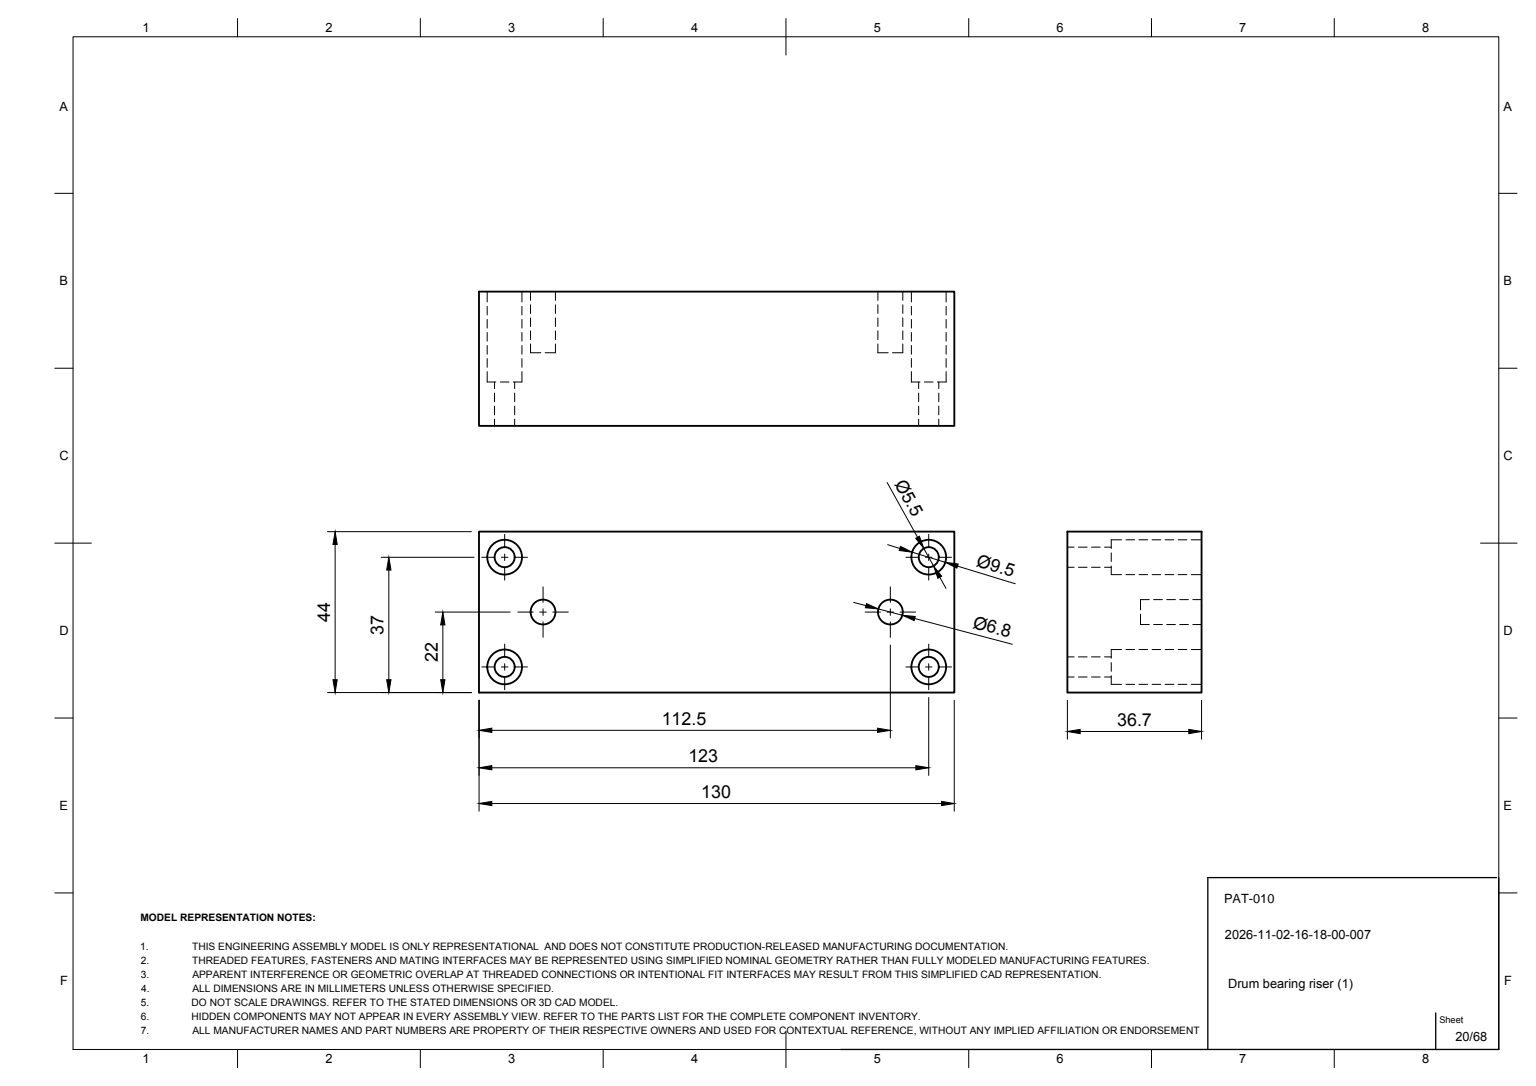
ISO-10303-21;
HEADER;
/* Generated by software containing ST-Developer
 * from STEP Tools, Inc. (www.steptools.com) 
 */

FILE_DESCRIPTION(
/* description */ ('Belt conveyor head drive unit'),
/* implementation_level */ '2;1');

FILE_NAME(
/* name */ 'Drum bearing riser (1).step',
/* time_stamp */ '2026-10-28T03:26:19-07:00',
/* author */ (''),
/* organization */ (''),
/* preprocessor_version */ 'ST-DEVELOPER v20.2',
/* originating_system */ 'Autodesk Translation Framework v15.17.0.0',
/* authorisation */ '');

FILE_SCHEMA (('AUTOMOTIVE_DESIGN { 1 0 10303 214 3 1 1 }'));
ENDSEC;

DATA;
#10=MECHANICAL_DESIGN_GEOMETRIC_PRESENTATION_REPRESENTATION('',(#866),#27069);
#728=SHAPE_REPRESENTATION_RELATIONSHIP('SRR','None',#27372,#797);
#797=ADVANCED_BREP_SHAPE_REPRESENTATION('',(#951),#27014);
#866=STYLED_ITEM('',(#27797),#951);
#951=MANIFOLD_SOLID_BREP('Body1',#13731);
#1111=FACE_BOUND('',#2762,.T.);
#1112=FACE_BOUND('',#2766,.T.);
#1113=FACE_BOUND('',#2770,.T.);
#1114=FACE_BOUND('',#2774,.T.);
#1115=FACE_BOUND('',#2785,.T.);
#1116=FACE_BOUND('',#2786,.T.);
#1117=FACE_BOUND('',#2787,.T.);
#1118=FACE_BOUND('',#2788,.T.);
#1119=FACE_BOUND('',#2789,.T.);
#1120=FACE_BOUND('',#2790,.T.);
#1121=FACE_BOUND('',#2792,.T.);
#1122=FACE_BOUND('',#2793,.T.);
#1123=FACE_BOUND('',#2794,.T.);
#1124=FACE_BOUND('',#2795,.T.);
#1389=PLANE('',#15059);
#1390=PLANE('',#15066);
#1391=PLANE('',#15073);
#1392=PLANE('',#15080);
#1393=PLANE('',#15087);
#1394=PLANE('',#15091);
#1395=PLANE('',#15092);
#1396=PLANE('',#15093);
#1397=PLANE('',#15094);
#1398=PLANE('',#15095);
#1399=PLANE('',#15096);
#1400=PLANE('',#15097);
#1861=FACE_OUTER_BOUND('',#2760,.T.);
#1862=FACE_OUTER_BOUND('',#2761,.T.);
#1863=FACE_OUTER_BOUND('',#2763,.T.);
#1864=FACE_OUTER_BOUND('',#2764,.T.);
#1865=FACE_OUTER_BOUND('',#2765,.T.);
#1866=FACE_OUTER_BOUND('',#2767,.T.);
#1867=FACE_OUTER_BOUND('',#2768,.T.);
#1868=FACE_OUTER_BOUND('',#2769,.T.);
#1869=FACE_OUTER_BOUND('',#2771,.T.);
#1870=FACE_OUTER_BOUND('',#2772,.T.);
#1871=FACE_OUTER_BOUND('',#2773,.T.);
#1872=FACE_OUTER_BOUND('',#2775,.T.);
#1873=FACE_OUTER_BOUND('',#2776,.T.);
#1874=FACE_OUTER_BOUND('',#2777,.T.);
#1875=FACE_OUTER_BOUND('',#2778,.T.);
#1876=FACE_OUTER_BOUND('',#2779,.T.);
#1877=FACE_OUTER_BOUND('',#2780,.T.);
#1878=FACE_OUTER_BOUND('',#2781,.T.);
#1879=FACE_OUTER_BOUND('',#2782,.T.);
#1880=FACE_OUTER_BOUND('',#2783,.T.);
#1881=FACE_OUTER_BOUND('',#2784,.T.);
#1882=FACE_OUTER_BOUND('',#2791,.T.);
#2760=EDGE_LOOP('',(#9972,#9973,#9974,#9975));
#2761=EDGE_LOOP('',(#9976));
#2762=EDGE_LOOP('',(#9977));
#2763=EDGE_LOOP('',(#9978,#9979,#9980,#9981));
#2764=EDGE_LOOP('',(#9982,#9983,#9984,#9985));
#2765=EDGE_LOOP('',(#9986));
#2766=EDGE_LOOP('',(#9987));
#2767=EDGE_LOOP('',(#9988,#9989,#9990,#9991));
#2768=EDGE_LOOP('',(#9992,#9993,#9994,#9995));
#2769=EDGE_LOOP('',(#9996));
#2770=EDGE_LOOP('',(#9997));
#2771=EDGE_LOOP('',(#9998,#9999,#10000,#10001));
#2772=EDGE_LOOP('',(#10002,#10003,#10004,#10005));
#2773=EDGE_LOOP('',(#10006));
#2774=EDGE_LOOP('',(#10007));
#2775=EDGE_LOOP('',(#10008,#10009,#10010,#10011));
#2776=EDGE_LOOP('',(#10012,#10013,#10014,#10015));
#2777=EDGE_LOOP('',(#10016));
#2778=EDGE_LOOP('',(#10017,#10018,#10019,#10020));
#2779=EDGE_LOOP('',(#10021));
#2780=EDGE_LOOP('',(#10022,#10023,#10024,#10025));
#2781=EDGE_LOOP('',(#10026,#10027,#10028,#10029));
#2782=EDGE_LOOP('',(#10030,#10031,#10032,#10033));
#2783=EDGE_LOOP('',(#10034,#10035,#10036,#10037));
#2784=EDGE_LOOP('',(#10038,#10039,#10040,#10041));
#2785=EDGE_LOOP('',(#10042));
#2786=EDGE_LOOP('',(#10043));
#2787=EDGE_LOOP('',(#10044));
#2788=EDGE_LOOP('',(#10045));
#2789=EDGE_LOOP('',(#10046));
#2790=EDGE_LOOP('',(#10047));
#2791=EDGE_LOOP('',(#10048,#10049,#10050,#10051));
#2792=EDGE_LOOP('',(#10052));
#2793=EDGE_LOOP('',(#10053));
#2794=EDGE_LOOP('',(#10054));
#2795=EDGE_LOOP('',(#10055));
#3761=LINE('',#22069,#4553);
#3762=LINE('',#22077,#4554);
#3763=LINE('',#22082,#4555);
#3764=LINE('',#22090,#4556);
#3765=LINE('',#22095,#4557);
#3766=LINE('',#22103,#4558);
#3767=LINE('',#22108,#4559);
#3768=LINE('',#22116,#4560);
#3769=LINE('',#22121,#4561);
#3770=LINE('',#22128,#4562);
#3771=LINE('',#22134,#4563);
#3772=LINE('',#22136,#4564);
#3773=LINE('',#22138,#4565);
#3774=LINE('',#22139,#4566);
#3775=LINE('',#22142,#4567);
#3776=LINE('',#22144,#4568);
#3777=LINE('',#22145,#4569);
#3778=LINE('',#22148,#4570);
#3779=LINE('',#22150,#4571);
#3780=LINE('',#22151,#4572);
#3781=LINE('',#22153,#4573);
#3782=LINE('',#22154,#4574);
#4553=VECTOR('',#17689,0.475);
#4554=VECTOR('',#17700,0.275);
#4555=VECTOR('',#17705,0.475);
#4556=VECTOR('',#17716,0.275);
#4557=VECTOR('',#17721,0.475);
#4558=VECTOR('',#17732,0.275);
#4559=VECTOR('',#17737,0.475);
#4560=VECTOR('',#17748,0.275);
#4561=VECTOR('',#17753,0.34);
#4562=VECTOR('',#17762,0.34);
#4563=VECTOR('',#17769,1.);
#4564=VECTOR('',#17770,1.);
#4565=VECTOR('',#17771,1.);
#4566=VECTOR('',#17772,1.);
#4567=VECTOR('',#17775,1.);
#4568=VECTOR('',#17776,1.);
#4569=VECTOR('',#17777,1.);
#4570=VECTOR('',#17780,1.);
#4571=VECTOR('',#17781,1.);
#4572=VECTOR('',#17782,1.);
#4573=VECTOR('',#17785,1.);
#4574=VECTOR('',#17786,1.);
#5326=CIRCLE('',#15057,0.475);
#5327=CIRCLE('',#15058,0.475);
#5328=CIRCLE('',#15060,0.275);
#5329=CIRCLE('',#15062,0.275);
#5330=CIRCLE('',#15064,0.475);
#5331=CIRCLE('',#15065,0.475);
#5332=CIRCLE('',#15067,0.275);
#5333=CIRCLE('',#15069,0.275);
#5334=CIRCLE('',#15071,0.475);
#5335=CIRCLE('',#15072,0.475);
#5336=CIRCLE('',#15074,0.275);
#5337=CIRCLE('',#15076,0.275);
#5338=CIRCLE('',#15078,0.475);
#5339=CIRCLE('',#15079,0.475);
#5340=CIRCLE('',#15081,0.275);
#5341=CIRCLE('',#15083,0.275);
#5342=CIRCLE('',#15085,0.34);
#5343=CIRCLE('',#15086,0.34);
#5344=CIRCLE('',#15089,0.34);
#5345=CIRCLE('',#15090,0.34);
#6291=VERTEX_POINT('',#22066);
#6292=VERTEX_POINT('',#22068);
#6293=VERTEX_POINT('',#22072);
#6294=VERTEX_POINT('',#22075);
#6295=VERTEX_POINT('',#22079);
#6296=VERTEX_POINT('',#22081);
#6297=VERTEX_POINT('',#22085);
#6298=VERTEX_POINT('',#22088);
#6299=VERTEX_POINT('',#22092);
#6300=VERTEX_POINT('',#22094);
#6301=VERTEX_POINT('',#22098);
#6302=VERTEX_POINT('',#22101);
#6303=VERTEX_POINT('',#22105);
#6304=VERTEX_POINT('',#22107);
#6305=VERTEX_POINT('',#22111);
#6306=VERTEX_POINT('',#22114);
#6307=VERTEX_POINT('',#22118);
#6308=VERTEX_POINT('',#22120);
#6309=VERTEX_POINT('',#22125);
#6310=VERTEX_POINT('',#22127);
#6311=VERTEX_POINT('',#22132);
#6312=VERTEX_POINT('',#22133);
#6313=VERTEX_POINT('',#22135);
#6314=VERTEX_POINT('',#22137);
#6315=VERTEX_POINT('',#22141);
#6316=VERTEX_POINT('',#22143);
#6317=VERTEX_POINT('',#22147);
#6318=VERTEX_POINT('',#22149);
#7678=EDGE_CURVE('',#6291,#6291,#5326,.T.);
#7679=EDGE_CURVE('',#6291,#6292,#3761,.T.);
#7680=EDGE_CURVE('',#6292,#6292,#5327,.T.);
#7681=EDGE_CURVE('',#6293,#6293,#5328,.T.);
#7682=EDGE_CURVE('',#6294,#6294,#5329,.T.);
#7683=EDGE_CURVE('',#6294,#6293,#3762,.T.);
#7684=EDGE_CURVE('',#6295,#6295,#5330,.T.);
#7685=EDGE_CURVE('',#6295,#6296,#3763,.T.);
#7686=EDGE_CURVE('',#6296,#6296,#5331,.T.);
#7687=EDGE_CURVE('',#6297,#6297,#5332,.T.);
#7688=EDGE_CURVE('',#6298,#6298,#5333,.T.);
#7689=EDGE_CURVE('',#6298,#6297,#3764,.T.);
#7690=EDGE_CURVE('',#6299,#6299,#5334,.T.);
#7691=EDGE_CURVE('',#6299,#6300,#3765,.T.);
#7692=EDGE_CURVE('',#6300,#6300,#5335,.T.);
#7693=EDGE_CURVE('',#6301,#6301,#5336,.T.);
#7694=EDGE_CURVE('',#6302,#6302,#5337,.T.);
#7695=EDGE_CURVE('',#6302,#6301,#3766,.T.);
#7696=EDGE_CURVE('',#6303,#6303,#5338,.T.);
#7697=EDGE_CURVE('',#6303,#6304,#3767,.T.);
#7698=EDGE_CURVE('',#6304,#6304,#5339,.T.);
#7699=EDGE_CURVE('',#6305,#6305,#5340,.T.);
#7700=EDGE_CURVE('',#6306,#6306,#5341,.T.);
#7701=EDGE_CURVE('',#6306,#6305,#3768,.T.);
#7702=EDGE_CURVE('',#6307,#6307,#5342,.T.);
#7703=EDGE_CURVE('',#6307,#6308,#3769,.T.);
#7704=EDGE_CURVE('',#6308,#6308,#5343,.T.);
#7705=EDGE_CURVE('',#6309,#6309,#5344,.T.);
#7706=EDGE_CURVE('',#6309,#6310,#3770,.T.);
#7707=EDGE_CURVE('',#6310,#6310,#5345,.T.);
#7708=EDGE_CURVE('',#6311,#6312,#3771,.T.);
#7709=EDGE_CURVE('',#6312,#6313,#3772,.T.);
#7710=EDGE_CURVE('',#6314,#6313,#3773,.T.);
#7711=EDGE_CURVE('',#6311,#6314,#3774,.T.);
#7712=EDGE_CURVE('',#6315,#6311,#3775,.T.);
#7713=EDGE_CURVE('',#6316,#6314,#3776,.T.);
#7714=EDGE_CURVE('',#6315,#6316,#3777,.T.);
#7715=EDGE_CURVE('',#6317,#6315,#3778,.T.);
#7716=EDGE_CURVE('',#6318,#6316,#3779,.T.);
#7717=EDGE_CURVE('',#6317,#6318,#3780,.T.);
#7718=EDGE_CURVE('',#6312,#6317,#3781,.T.);
#7719=EDGE_CURVE('',#6313,#6318,#3782,.T.);
#9972=ORIENTED_EDGE('',*,*,#7678,.F.);
#9973=ORIENTED_EDGE('',*,*,#7679,.T.);
#9974=ORIENTED_EDGE('',*,*,#7680,.F.);
#9975=ORIENTED_EDGE('',*,*,#7679,.F.);
#9976=ORIENTED_EDGE('',*,*,#7678,.T.);
#9977=ORIENTED_EDGE('',*,*,#7681,.F.);
#9978=ORIENTED_EDGE('',*,*,#7682,.F.);
#9979=ORIENTED_EDGE('',*,*,#7683,.T.);
#9980=ORIENTED_EDGE('',*,*,#7681,.T.);
#9981=ORIENTED_EDGE('',*,*,#7683,.F.);
#9982=ORIENTED_EDGE('',*,*,#7684,.F.);
#9983=ORIENTED_EDGE('',*,*,#7685,.T.);
#9984=ORIENTED_EDGE('',*,*,#7686,.F.);
#9985=ORIENTED_EDGE('',*,*,#7685,.F.);
#9986=ORIENTED_EDGE('',*,*,#7684,.T.);
#9987=ORIENTED_EDGE('',*,*,#7687,.F.);
#9988=ORIENTED_EDGE('',*,*,#7688,.F.);
#9989=ORIENTED_EDGE('',*,*,#7689,.T.);
#9990=ORIENTED_EDGE('',*,*,#7687,.T.);
#9991=ORIENTED_EDGE('',*,*,#7689,.F.);
#9992=ORIENTED_EDGE('',*,*,#7690,.F.);
#9993=ORIENTED_EDGE('',*,*,#7691,.T.);
#9994=ORIENTED_EDGE('',*,*,#7692,.F.);
#9995=ORIENTED_EDGE('',*,*,#7691,.F.);
#9996=ORIENTED_EDGE('',*,*,#7690,.T.);
#9997=ORIENTED_EDGE('',*,*,#7693,.F.);
#9998=ORIENTED_EDGE('',*,*,#7694,.F.);
#9999=ORIENTED_EDGE('',*,*,#7695,.T.);
#10000=ORIENTED_EDGE('',*,*,#7693,.T.);
#10001=ORIENTED_EDGE('',*,*,#7695,.F.);
#10002=ORIENTED_EDGE('',*,*,#7696,.F.);
#10003=ORIENTED_EDGE('',*,*,#7697,.T.);
#10004=ORIENTED_EDGE('',*,*,#7698,.F.);
#10005=ORIENTED_EDGE('',*,*,#7697,.F.);
#10006=ORIENTED_EDGE('',*,*,#7696,.T.);
#10007=ORIENTED_EDGE('',*,*,#7699,.F.);
#10008=ORIENTED_EDGE('',*,*,#7700,.F.);
#10009=ORIENTED_EDGE('',*,*,#7701,.T.);
#10010=ORIENTED_EDGE('',*,*,#7699,.T.);
#10011=ORIENTED_EDGE('',*,*,#7701,.F.);
#10012=ORIENTED_EDGE('',*,*,#7702,.F.);
#10013=ORIENTED_EDGE('',*,*,#7703,.T.);
#10014=ORIENTED_EDGE('',*,*,#7704,.F.);
#10015=ORIENTED_EDGE('',*,*,#7703,.F.);
#10016=ORIENTED_EDGE('',*,*,#7702,.T.);
#10017=ORIENTED_EDGE('',*,*,#7705,.F.);
#10018=ORIENTED_EDGE('',*,*,#7706,.T.);
#10019=ORIENTED_EDGE('',*,*,#7707,.F.);
#10020=ORIENTED_EDGE('',*,*,#7706,.F.);
#10021=ORIENTED_EDGE('',*,*,#7705,.T.);
#10022=ORIENTED_EDGE('',*,*,#7708,.T.);
#10023=ORIENTED_EDGE('',*,*,#7709,.T.);
#10024=ORIENTED_EDGE('',*,*,#7710,.F.);
#10025=ORIENTED_EDGE('',*,*,#7711,.F.);
#10026=ORIENTED_EDGE('',*,*,#7712,.T.);
#10027=ORIENTED_EDGE('',*,*,#7711,.T.);
#10028=ORIENTED_EDGE('',*,*,#7713,.F.);
#10029=ORIENTED_EDGE('',*,*,#7714,.F.);
#10030=ORIENTED_EDGE('',*,*,#7715,.T.);
#10031=ORIENTED_EDGE('',*,*,#7714,.T.);
#10032=ORIENTED_EDGE('',*,*,#7716,.F.);
#10033=ORIENTED_EDGE('',*,*,#7717,.F.);
#10034=ORIENTED_EDGE('',*,*,#7718,.T.);
#10035=ORIENTED_EDGE('',*,*,#7717,.T.);
#10036=ORIENTED_EDGE('',*,*,#7719,.F.);
#10037=ORIENTED_EDGE('',*,*,#7709,.F.);
#10038=ORIENTED_EDGE('',*,*,#7719,.T.);
#10039=ORIENTED_EDGE('',*,*,#7716,.T.);
#10040=ORIENTED_EDGE('',*,*,#7713,.T.);
#10041=ORIENTED_EDGE('',*,*,#7710,.T.);
#10042=ORIENTED_EDGE('',*,*,#7680,.T.);
#10043=ORIENTED_EDGE('',*,*,#7686,.T.);
#10044=ORIENTED_EDGE('',*,*,#7692,.T.);
#10045=ORIENTED_EDGE('',*,*,#7698,.T.);
#10046=ORIENTED_EDGE('',*,*,#7704,.T.);
#10047=ORIENTED_EDGE('',*,*,#7707,.T.);
#10048=ORIENTED_EDGE('',*,*,#7718,.F.);
#10049=ORIENTED_EDGE('',*,*,#7708,.F.);
#10050=ORIENTED_EDGE('',*,*,#7712,.F.);
#10051=ORIENTED_EDGE('',*,*,#7715,.F.);
#10052=ORIENTED_EDGE('',*,*,#7682,.T.);
#10053=ORIENTED_EDGE('',*,*,#7688,.T.);
#10054=ORIENTED_EDGE('',*,*,#7694,.T.);
#10055=ORIENTED_EDGE('',*,*,#7700,.T.);
#12648=CYLINDRICAL_SURFACE('',#15056,0.475);
#12649=CYLINDRICAL_SURFACE('',#15061,0.275);
#12650=CYLINDRICAL_SURFACE('',#15063,0.475);
#12651=CYLINDRICAL_SURFACE('',#15068,0.275);
#12652=CYLINDRICAL_SURFACE('',#15070,0.475);
#12653=CYLINDRICAL_SURFACE('',#15075,0.275);
#12654=CYLINDRICAL_SURFACE('',#15077,0.475);
#12655=CYLINDRICAL_SURFACE('',#15082,0.275);
#12656=CYLINDRICAL_SURFACE('',#15084,0.34);
#12657=CYLINDRICAL_SURFACE('',#15088,0.34);
#13140=ADVANCED_FACE('',(#1861),#12648,.F.);
#13141=ADVANCED_FACE('',(#1862,#1111),#1389,.T.);
#13142=ADVANCED_FACE('',(#1863),#12649,.F.);
#13143=ADVANCED_FACE('',(#1864),#12650,.F.);
#13144=ADVANCED_FACE('',(#1865,#1112),#1390,.T.);
#13145=ADVANCED_FACE('',(#1866),#12651,.F.);
#13146=ADVANCED_FACE('',(#1867),#12652,.F.);
#13147=ADVANCED_FACE('',(#1868,#1113),#1391,.T.);
#13148=ADVANCED_FACE('',(#1869),#12653,.F.);
#13149=ADVANCED_FACE('',(#1870),#12654,.F.);
#13150=ADVANCED_FACE('',(#1871,#1114),#1392,.T.);
#13151=ADVANCED_FACE('',(#1872),#12655,.F.);
#13152=ADVANCED_FACE('',(#1873),#12656,.F.);
#13153=ADVANCED_FACE('',(#1874),#1393,.T.);
#13154=ADVANCED_FACE('',(#1875),#12657,.F.);
#13155=ADVANCED_FACE('',(#1876),#1394,.T.);
#13156=ADVANCED_FACE('',(#1877),#1395,.T.);
#13157=ADVANCED_FACE('',(#1878),#1396,.T.);
#13158=ADVANCED_FACE('',(#1879),#1397,.T.);
#13159=ADVANCED_FACE('',(#1880),#1398,.T.);
#13160=ADVANCED_FACE('',(#1881,#1115,#1116,#1117,#1118,#1119,#1120),#1399,
 .T.);
#13161=ADVANCED_FACE('',(#1882,#1121,#1122,#1123,#1124),#1400,.F.);
#13731=CLOSED_SHELL('',(#13140,#13141,#13142,#13143,#13144,#13145,#13146,
#13147,#13148,#13149,#13150,#13151,#13152,#13153,#13154,#13155,#13156,#13157,
#13158,#13159,#13160,#13161));
#15055=AXIS2_PLACEMENT_3D('',#22064,#17683,#17684);
#15056=AXIS2_PLACEMENT_3D('',#22065,#17685,#17686);
#15057=AXIS2_PLACEMENT_3D('',#22067,#17687,#17688);
#15058=AXIS2_PLACEMENT_3D('',#22070,#17690,#17691);
#15059=AXIS2_PLACEMENT_3D('',#22071,#17692,#17693);
#15060=AXIS2_PLACEMENT_3D('',#22073,#17694,#17695);
#15061=AXIS2_PLACEMENT_3D('',#22074,#17696,#17697);
#15062=AXIS2_PLACEMENT_3D('',#22076,#17698,#17699);
#15063=AXIS2_PLACEMENT_3D('',#22078,#17701,#17702);
#15064=AXIS2_PLACEMENT_3D('',#22080,#17703,#17704);
#15065=AXIS2_PLACEMENT_3D('',#22083,#17706,#17707);
#15066=AXIS2_PLACEMENT_3D('',#22084,#17708,#17709);
#15067=AXIS2_PLACEMENT_3D('',#22086,#17710,#17711);
#15068=AXIS2_PLACEMENT_3D('',#22087,#17712,#17713);
#15069=AXIS2_PLACEMENT_3D('',#22089,#17714,#17715);
#15070=AXIS2_PLACEMENT_3D('',#22091,#17717,#17718);
#15071=AXIS2_PLACEMENT_3D('',#22093,#17719,#17720);
#15072=AXIS2_PLACEMENT_3D('',#22096,#17722,#17723);
#15073=AXIS2_PLACEMENT_3D('',#22097,#17724,#17725);
#15074=AXIS2_PLACEMENT_3D('',#22099,#17726,#17727);
#15075=AXIS2_PLACEMENT_3D('',#22100,#17728,#17729);
#15076=AXIS2_PLACEMENT_3D('',#22102,#17730,#17731);
#15077=AXIS2_PLACEMENT_3D('',#22104,#17733,#17734);
#15078=AXIS2_PLACEMENT_3D('',#22106,#17735,#17736);
#15079=AXIS2_PLACEMENT_3D('',#22109,#17738,#17739);
#15080=AXIS2_PLACEMENT_3D('',#22110,#17740,#17741);
#15081=AXIS2_PLACEMENT_3D('',#22112,#17742,#17743);
#15082=AXIS2_PLACEMENT_3D('',#22113,#17744,#17745);
#15083=AXIS2_PLACEMENT_3D('',#22115,#17746,#17747);
#15084=AXIS2_PLACEMENT_3D('',#22117,#17749,#17750);
#15085=AXIS2_PLACEMENT_3D('',#22119,#17751,#17752);
#15086=AXIS2_PLACEMENT_3D('',#22122,#17754,#17755);
#15087=AXIS2_PLACEMENT_3D('',#22123,#17756,#17757);
#15088=AXIS2_PLACEMENT_3D('',#22124,#17758,#17759);
#15089=AXIS2_PLACEMENT_3D('',#22126,#17760,#17761);
#15090=AXIS2_PLACEMENT_3D('',#22129,#17763,#17764);
#15091=AXIS2_PLACEMENT_3D('',#22130,#17765,#17766);
#15092=AXIS2_PLACEMENT_3D('',#22131,#17767,#17768);
#15093=AXIS2_PLACEMENT_3D('',#22140,#17773,#17774);
#15094=AXIS2_PLACEMENT_3D('',#22146,#17778,#17779);
#15095=AXIS2_PLACEMENT_3D('',#22152,#17783,#17784);
#15096=AXIS2_PLACEMENT_3D('',#22155,#17787,#17788);
#15097=AXIS2_PLACEMENT_3D('',#22156,#17789,#17790);
#17683=DIRECTION('axis',(0.,0.,1.));
#17684=DIRECTION('refdir',(1.,0.,0.));
#17685=DIRECTION('center_axis',(0.,0.,1.));
#17686=DIRECTION('ref_axis',(1.,0.,0.));
#17687=DIRECTION('center_axis',(0.,0.,1.));
#17688=DIRECTION('ref_axis',(1.,0.,0.));
#17689=DIRECTION('',(0.,0.,1.));
#17690=DIRECTION('center_axis',(0.,0.,-1.));
#17691=DIRECTION('ref_axis',(1.,0.,0.));
#17692=DIRECTION('center_axis',(0.,0.,1.));
#17693=DIRECTION('ref_axis',(1.,0.,0.));
#17694=DIRECTION('center_axis',(0.,0.,1.));
#17695=DIRECTION('ref_axis',(1.,0.,0.));
#17696=DIRECTION('center_axis',(0.,0.,1.));
#17697=DIRECTION('ref_axis',(1.,0.,0.));
#17698=DIRECTION('center_axis',(0.,0.,1.));
#17699=DIRECTION('ref_axis',(1.,0.,0.));
#17700=DIRECTION('',(0.,0.,1.));
#17701=DIRECTION('center_axis',(0.,0.,1.));
#17702=DIRECTION('ref_axis',(1.,0.,0.));
#17703=DIRECTION('center_axis',(0.,0.,1.));
#17704=DIRECTION('ref_axis',(1.,0.,0.));
#17705=DIRECTION('',(0.,0.,1.));
#17706=DIRECTION('center_axis',(0.,0.,-1.));
#17707=DIRECTION('ref_axis',(1.,0.,0.));
#17708=DIRECTION('center_axis',(0.,0.,1.));
#17709=DIRECTION('ref_axis',(1.,0.,0.));
#17710=DIRECTION('center_axis',(0.,0.,1.));
#17711=DIRECTION('ref_axis',(1.,0.,0.));
#17712=DIRECTION('center_axis',(0.,0.,1.));
#17713=DIRECTION('ref_axis',(1.,0.,0.));
#17714=DIRECTION('center_axis',(0.,0.,1.));
#17715=DIRECTION('ref_axis',(1.,0.,0.));
#17716=DIRECTION('',(0.,0.,1.));
#17717=DIRECTION('center_axis',(0.,0.,1.));
#17718=DIRECTION('ref_axis',(1.,0.,0.));
#17719=DIRECTION('center_axis',(0.,0.,1.));
#17720=DIRECTION('ref_axis',(1.,0.,0.));
#17721=DIRECTION('',(0.,0.,1.));
#17722=DIRECTION('center_axis',(0.,0.,-1.));
#17723=DIRECTION('ref_axis',(1.,0.,0.));
#17724=DIRECTION('center_axis',(0.,0.,1.));
#17725=DIRECTION('ref_axis',(1.,0.,0.));
#17726=DIRECTION('center_axis',(0.,0.,1.));
#17727=DIRECTION('ref_axis',(1.,0.,0.));
#17728=DIRECTION('center_axis',(0.,0.,1.));
#17729=DIRECTION('ref_axis',(1.,0.,0.));
#17730=DIRECTION('center_axis',(0.,0.,1.));
#17731=DIRECTION('ref_axis',(1.,0.,0.));
#17732=DIRECTION('',(0.,0.,1.));
#17733=DIRECTION('center_axis',(0.,0.,1.));
#17734=DIRECTION('ref_axis',(1.,0.,0.));
#17735=DIRECTION('center_axis',(0.,0.,1.));
#17736=DIRECTION('ref_axis',(1.,0.,0.));
#17737=DIRECTION('',(0.,0.,1.));
#17738=DIRECTION('center_axis',(0.,0.,-1.));
#17739=DIRECTION('ref_axis',(1.,0.,0.));
#17740=DIRECTION('center_axis',(0.,0.,1.));
#17741=DIRECTION('ref_axis',(1.,0.,0.));
#17742=DIRECTION('center_axis',(0.,0.,1.));
#17743=DIRECTION('ref_axis',(1.,0.,0.));
#17744=DIRECTION('center_axis',(0.,0.,1.));
#17745=DIRECTION('ref_axis',(1.,0.,0.));
#17746=DIRECTION('center_axis',(0.,0.,1.));
#17747=DIRECTION('ref_axis',(1.,0.,0.));
#17748=DIRECTION('',(0.,0.,1.));
#17749=DIRECTION('center_axis',(0.,0.,1.));
#17750=DIRECTION('ref_axis',(1.,0.,0.));
#17751=DIRECTION('center_axis',(0.,0.,1.));
#17752=DIRECTION('ref_axis',(1.,0.,0.));
#17753=DIRECTION('',(0.,0.,1.));
#17754=DIRECTION('center_axis',(0.,0.,-1.));
#17755=DIRECTION('ref_axis',(1.,0.,0.));
#17756=DIRECTION('center_axis',(0.,0.,1.));
#17757=DIRECTION('ref_axis',(1.,0.,0.));
#17758=DIRECTION('center_axis',(0.,0.,1.));
#17759=DIRECTION('ref_axis',(1.,0.,0.));
#17760=DIRECTION('center_axis',(0.,0.,1.));
#17761=DIRECTION('ref_axis',(1.,0.,0.));
#17762=DIRECTION('',(0.,0.,1.));
#17763=DIRECTION('center_axis',(0.,0.,-1.));
#17764=DIRECTION('ref_axis',(1.,0.,0.));
#17765=DIRECTION('center_axis',(0.,0.,1.));
#17766=DIRECTION('ref_axis',(1.,0.,0.));
#17767=DIRECTION('center_axis',(0.,1.,0.));
#17768=DIRECTION('ref_axis',(-1.,0.,0.));
#17769=DIRECTION('',(-1.,0.,0.));
#17770=DIRECTION('',(0.,0.,1.));
#17771=DIRECTION('',(-1.,0.,0.));
#17772=DIRECTION('',(0.,0.,1.));
#17773=DIRECTION('center_axis',(1.,0.,0.));
#17774=DIRECTION('ref_axis',(0.,1.,0.));
#17775=DIRECTION('',(0.,1.,0.));
#17776=DIRECTION('',(0.,1.,0.));
#17777=DIRECTION('',(0.,0.,1.));
#17778=DIRECTION('center_axis',(0.,-1.,0.));
#17779=DIRECTION('ref_axis',(1.,0.,0.));
#17780=DIRECTION('',(1.,0.,0.));
#17781=DIRECTION('',(1.,0.,0.));
#17782=DIRECTION('',(0.,0.,1.));
#17783=DIRECTION('center_axis',(-1.,0.,0.));
#17784=DIRECTION('ref_axis',(0.,-1.,0.));
#17785=DIRECTION('',(0.,-1.,0.));
#17786=DIRECTION('',(0.,-1.,0.));
#17787=DIRECTION('center_axis',(0.,0.,1.));
#17788=DIRECTION('ref_axis',(1.,0.,0.));
#17789=DIRECTION('center_axis',(0.,0.,1.));
#17790=DIRECTION('ref_axis',(1.,0.,0.));
#22064=CARTESIAN_POINT('',(0.,0.,0.));
#22065=CARTESIAN_POINT('Origin',(12.7709100301812,41.5,1.2));
#22066=CARTESIAN_POINT('',(12.2959100301812,41.5,1.2));
#22067=CARTESIAN_POINT('Origin',(12.7709100301812,41.5,1.2));
#22068=CARTESIAN_POINT('',(12.2959100301812,41.5,3.67));
#22069=CARTESIAN_POINT('',(12.2959100301812,41.5,1.2));
#22070=CARTESIAN_POINT('Origin',(12.7709100301812,41.5,3.67));
#22071=CARTESIAN_POINT('Origin',(12.7709100301812,41.5,1.2));
#22072=CARTESIAN_POINT('',(12.4959100301812,41.5,1.2));
#22073=CARTESIAN_POINT('Origin',(12.7709100301812,41.5,1.2));
#22074=CARTESIAN_POINT('Origin',(12.7709100301812,41.5,-0.1));
#22075=CARTESIAN_POINT('',(12.4959100301812,41.5,0.));
#22076=CARTESIAN_POINT('Origin',(12.7709100301812,41.5,0.));
#22077=CARTESIAN_POINT('',(12.4959100301812,41.5,-0.1));
#22078=CARTESIAN_POINT('Origin',(12.7709100301812,38.5,1.2));
#22079=CARTESIAN_POINT('',(12.2959100301812,38.5,1.2));
#22080=CARTESIAN_POINT('Origin',(12.7709100301812,38.5,1.2));
#22081=CARTESIAN_POINT('',(12.2959100301812,38.5,3.67));
#22082=CARTESIAN_POINT('',(12.2959100301812,38.5,1.2));
#22083=CARTESIAN_POINT('Origin',(12.7709100301812,38.5,3.67));
#22084=CARTESIAN_POINT('Origin',(12.7709100301812,38.5,1.2));
#22085=CARTESIAN_POINT('',(12.4959100301812,38.5,1.2));
#22086=CARTESIAN_POINT('Origin',(12.7709100301812,38.5,1.2));
#22087=CARTESIAN_POINT('Origin',(12.7709100301812,38.5,-0.1));
#22088=CARTESIAN_POINT('',(12.4959100301812,38.5,0.));
#22089=CARTESIAN_POINT('Origin',(12.7709100301812,38.5,0.));
#22090=CARTESIAN_POINT('',(12.4959100301812,38.5,-0.1));
#22091=CARTESIAN_POINT('Origin',(1.17091003018116,41.5,1.2));
#22092=CARTESIAN_POINT('',(0.695910030181156,41.5,1.2));
#22093=CARTESIAN_POINT('Origin',(1.17091003018116,41.5,1.2));
#22094=CARTESIAN_POINT('',(0.695910030181156,41.5,3.67));
#22095=CARTESIAN_POINT('',(0.695910030181156,41.5,1.2));
#22096=CARTESIAN_POINT('Origin',(1.17091003018116,41.5,3.67));
#22097=CARTESIAN_POINT('Origin',(1.17091003018116,41.5,1.2));
#22098=CARTESIAN_POINT('',(0.895910030181156,41.5,1.2));
#22099=CARTESIAN_POINT('Origin',(1.17091003018116,41.5,1.2));
#22100=CARTESIAN_POINT('Origin',(1.17091003018116,41.5,-0.1));
#22101=CARTESIAN_POINT('',(0.895910030181156,41.5,0.));
#22102=CARTESIAN_POINT('Origin',(1.17091003018116,41.5,0.));
#22103=CARTESIAN_POINT('',(0.895910030181156,41.5,-0.1));
#22104=CARTESIAN_POINT('Origin',(1.17091003018116,38.5,1.2));
#22105=CARTESIAN_POINT('',(0.695910030181156,38.5,1.2));
#22106=CARTESIAN_POINT('Origin',(1.17091003018116,38.5,1.2));
#22107=CARTESIAN_POINT('',(0.695910030181156,38.5,3.67));
#22108=CARTESIAN_POINT('',(0.695910030181156,38.5,1.2));
#22109=CARTESIAN_POINT('Origin',(1.17091003018116,38.5,3.67));
#22110=CARTESIAN_POINT('Origin',(1.17091003018116,38.5,1.2));
#22111=CARTESIAN_POINT('',(0.895910030181156,38.5,1.2));
#22112=CARTESIAN_POINT('Origin',(1.17091003018116,38.5,1.2));
#22113=CARTESIAN_POINT('Origin',(1.17091003018116,38.5,-0.1));
#22114=CARTESIAN_POINT('',(0.895910030181156,38.5,0.));
#22115=CARTESIAN_POINT('Origin',(1.17091003018116,38.5,0.));
#22116=CARTESIAN_POINT('',(0.895910030181156,38.5,-0.1));
#22117=CARTESIAN_POINT('Origin',(2.22091003018116,40.,2.));
#22118=CARTESIAN_POINT('',(1.88091003018116,40.,2.));
#22119=CARTESIAN_POINT('Origin',(2.22091003018116,40.,2.));
#22120=CARTESIAN_POINT('',(1.88091003018116,40.,3.67));
#22121=CARTESIAN_POINT('',(1.88091003018116,40.,2.));
#22122=CARTESIAN_POINT('Origin',(2.22091003018116,40.,3.67));
#22123=CARTESIAN_POINT('Origin',(2.22091003018116,40.,2.));
#22124=CARTESIAN_POINT('Origin',(11.7209100301812,40.,2.));
#22125=CARTESIAN_POINT('',(11.3809100301812,40.,2.));
#22126=CARTESIAN_POINT('Origin',(11.7209100301812,40.,2.));
#22127=CARTESIAN_POINT('',(11.3809100301812,40.,3.67));
#22128=CARTESIAN_POINT('',(11.3809100301812,40.,2.));
#22129=CARTESIAN_POINT('Origin',(11.7209100301812,40.,3.67));
#22130=CARTESIAN_POINT('Origin',(11.7209100301812,40.,2.));
#22131=CARTESIAN_POINT('Origin',(13.4709100301812,42.2,0.));
#22132=CARTESIAN_POINT('',(13.4709100301812,42.2,0.));
#22133=CARTESIAN_POINT('',(0.470910030181156,42.2,0.));
#22134=CARTESIAN_POINT('',(13.4709100301812,42.2,0.));
#22135=CARTESIAN_POINT('',(0.470910030181156,42.2,3.67));
#22136=CARTESIAN_POINT('',(0.470910030181156,42.2,0.));
#22137=CARTESIAN_POINT('',(13.4709100301812,42.2,3.67));
#22138=CARTESIAN_POINT('',(13.4709100301812,42.2,3.67));
#22139=CARTESIAN_POINT('',(13.4709100301812,42.2,0.));
#22140=CARTESIAN_POINT('Origin',(13.4709100301812,37.8,0.));
#22141=CARTESIAN_POINT('',(13.4709100301812,37.8,0.));
#22142=CARTESIAN_POINT('',(13.4709100301812,37.8,0.));
#22143=CARTESIAN_POINT('',(13.4709100301812,37.8,3.67));
#22144=CARTESIAN_POINT('',(13.4709100301812,37.8,3.67));
#22145=CARTESIAN_POINT('',(13.4709100301812,37.8,0.));
#22146=CARTESIAN_POINT('Origin',(0.470910030181156,37.8,0.));
#22147=CARTESIAN_POINT('',(0.470910030181156,37.8,0.));
#22148=CARTESIAN_POINT('',(0.470910030181156,37.8,0.));
#22149=CARTESIAN_POINT('',(0.470910030181156,37.8,3.67));
#22150=CARTESIAN_POINT('',(0.470910030181156,37.8,3.67));
#22151=CARTESIAN_POINT('',(0.470910030181156,37.8,0.));
#22152=CARTESIAN_POINT('Origin',(0.470910030181156,42.2,0.));
#22153=CARTESIAN_POINT('',(0.470910030181156,42.2,0.));
#22154=CARTESIAN_POINT('',(0.470910030181156,42.2,3.67));
#22155=CARTESIAN_POINT('Origin',(6.97091003018116,40.,3.67));
#22156=CARTESIAN_POINT('Origin',(6.97091003018116,40.,0.));
#26937=UNCERTAINTY_MEASURE_WITH_UNIT(LENGTH_MEASURE(0.001),#27070,
'DISTANCE_ACCURACY_VALUE',
'Maximum model space distance between geometric entities at asserted c
onnectivities');
#26992=UNCERTAINTY_MEASURE_WITH_UNIT(LENGTH_MEASURE(0.001),#27070,
'DISTANCE_ACCURACY_VALUE',
'Maximum model space distance between geometric entities at asserted c
onnectivities');
#27014=(
GEOMETRIC_REPRESENTATION_CONTEXT(3)
GLOBAL_UNCERTAINTY_ASSIGNED_CONTEXT((#26937))
GLOBAL_UNIT_ASSIGNED_CONTEXT((#27070,#27072,#27073))
REPRESENTATION_CONTEXT('','3D')
);
#27069=(
GEOMETRIC_REPRESENTATION_CONTEXT(3)
GLOBAL_UNCERTAINTY_ASSIGNED_CONTEXT((#26992))
GLOBAL_UNIT_ASSIGNED_CONTEXT((#27070,#27072,#27073))
REPRESENTATION_CONTEXT('','3D')
);
#27070=(
LENGTH_UNIT()
NAMED_UNIT(*)
SI_UNIT(.CENTI.,.METRE.)
);
#27072=(
NAMED_UNIT(*)
PLANE_ANGLE_UNIT()
SI_UNIT($,.RADIAN.)
);
#27073=(
NAMED_UNIT(*)
SI_UNIT($,.STERADIAN.)
SOLID_ANGLE_UNIT()
);
#27095=SHAPE_DEFINITION_REPRESENTATION(#27171,#27372);
#27171=PRODUCT_DEFINITION_SHAPE('',$,#27449);
#27372=SHAPE_REPRESENTATION('',(#15055),#27014);
#27427=PRODUCT_DEFINITION_CONTEXT('part definition',#27657,'design');
#27449=PRODUCT_DEFINITION('Drum bearing riser (1)',
'Drum bearing riser (1)',#27525,#27427);
#27525=PRODUCT_DEFINITION_FORMATION('',$,#27680);
#27657=APPLICATION_CONTEXT(
'Core Data for Automotive Mechanical Design Process');
#27658=PRODUCT_CONTEXT('part definition',#27657,'mechanical');
#27680=PRODUCT('Drum bearing riser (1)','Drum bearing riser (1)',
'Drum bearing riser (1)',(#27658));
#27791=COLOUR_RGB('Grey',0.48,0.52,0.57);
#27792=FILL_AREA_STYLE_COLOUR('',#27791);
#27793=FILL_AREA_STYLE('',(#27792));
#27794=SURFACE_STYLE_FILL_AREA(#27793);
#27795=SURFACE_SIDE_STYLE('',(#27794));
#27796=SURFACE_STYLE_USAGE(.BOTH.,#27795);
#27797=PRESENTATION_STYLE_ASSIGNMENT((#27796));
ENDSEC;
END-ISO-10303-21;
